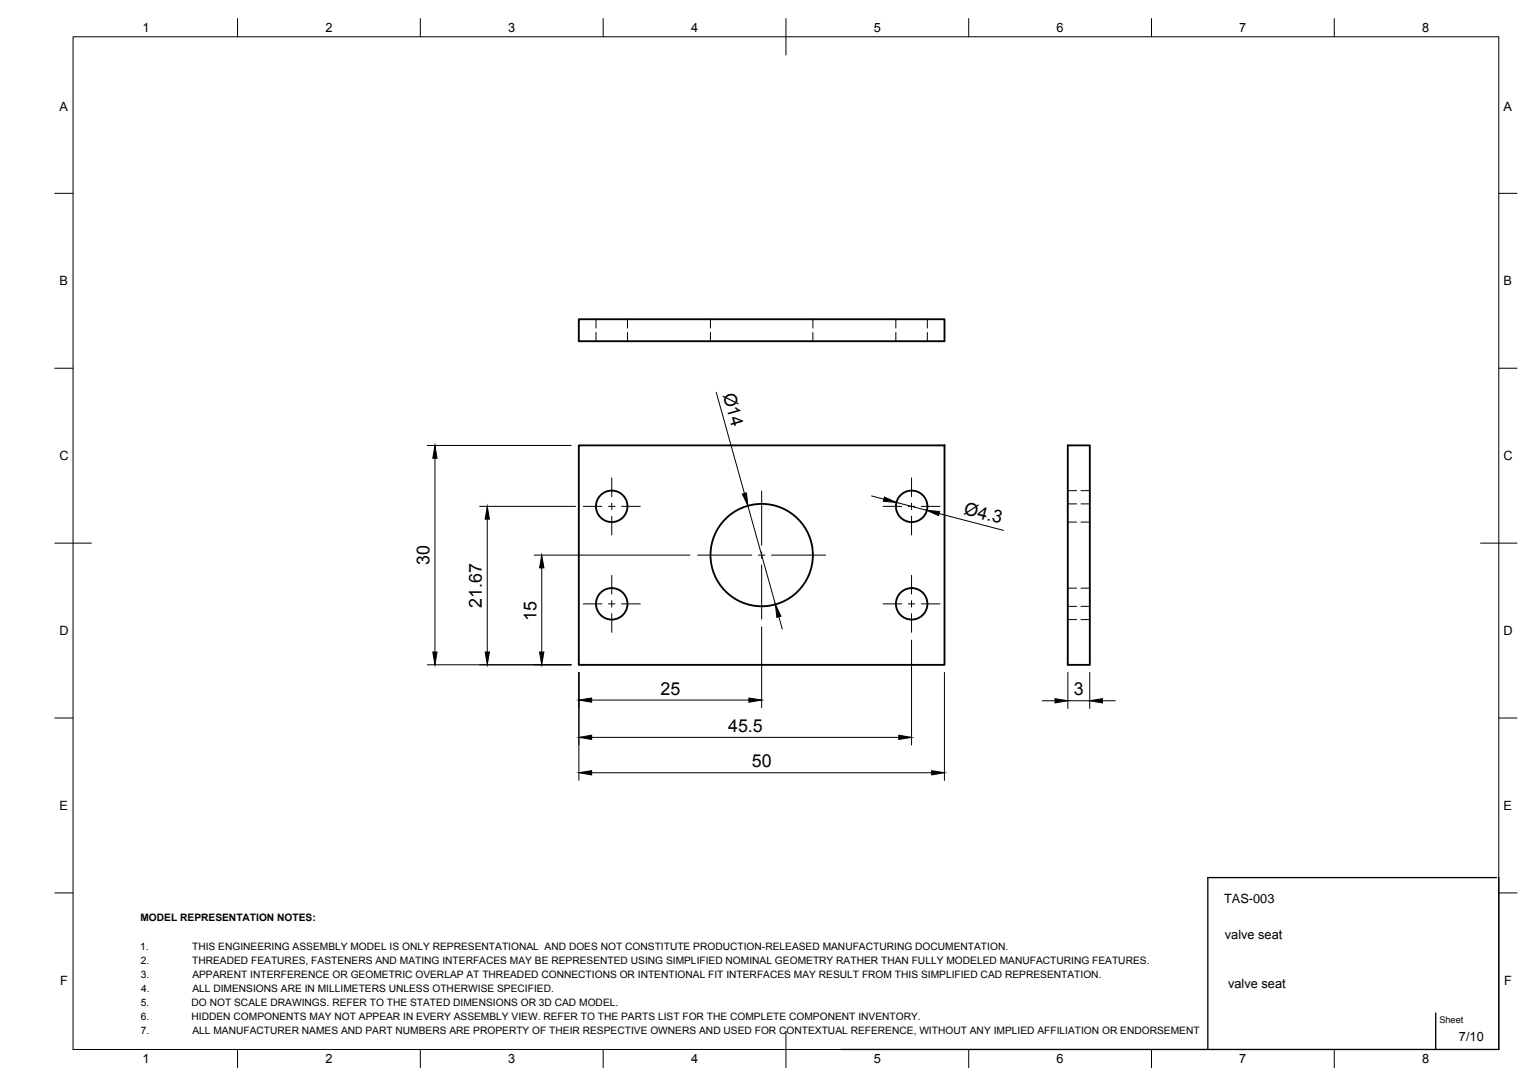
ISO-10303-21;
HEADER;
/* Generated by software containing ST-Developer
 * from STEP Tools, Inc. (www.steptools.com) 
 */

FILE_DESCRIPTION(
/* description */ ('STEP AP214'),
/* implementation_level */ '2;1');

FILE_NAME(
/* name */ 'valve seat.step',
/* time_stamp */ '2026-11-04T19:43:37-08:00',
/* author */ (''),
/* organization */ (''),
/* preprocessor_version */ 'ST-DEVELOPER v20.2',
/* originating_system */ 'Autodesk Translation Framework v15.17.0.0',
/* authorisation */ '');

FILE_SCHEMA (('AUTOMOTIVE_DESIGN { 1 0 10303 214 3 1 1 }'));
ENDSEC;

DATA;
#10=MECHANICAL_DESIGN_GEOMETRIC_PRESENTATION_REPRESENTATION('',(#119),#7627);
#101=SHAPE_REPRESENTATION_RELATIONSHIP('SRR','None',#7669,#110);
#110=ADVANCED_BREP_SHAPE_REPRESENTATION('',(#140),#7622);
#119=STYLED_ITEM('',(#7720),#140);
#140=MANIFOLD_SOLID_BREP('Body1',#2417);
#168=FACE_BOUND('',#518,.T.);
#169=FACE_BOUND('',#519,.T.);
#170=FACE_BOUND('',#520,.T.);
#171=FACE_BOUND('',#521,.T.);
#172=FACE_BOUND('',#522,.T.);
#173=FACE_BOUND('',#524,.T.);
#174=FACE_BOUND('',#525,.T.);
#175=FACE_BOUND('',#526,.T.);
#176=FACE_BOUND('',#527,.T.);
#177=FACE_BOUND('',#528,.T.);
#211=PLANE('',#2624);
#212=PLANE('',#2625);
#213=PLANE('',#2626);
#214=PLANE('',#2627);
#215=PLANE('',#2628);
#216=PLANE('',#2629);
#268=CYLINDRICAL_SURFACE('',#2609,2.15);
#269=CYLINDRICAL_SURFACE('',#2612,2.15);
#270=CYLINDRICAL_SURFACE('',#2615,2.15);
#271=CYLINDRICAL_SURFACE('',#2618,2.15);
#272=CYLINDRICAL_SURFACE('',#2621,7.);
#347=FACE_OUTER_BOUND('',#512,.T.);
#348=FACE_OUTER_BOUND('',#513,.T.);
#349=FACE_OUTER_BOUND('',#514,.T.);
#350=FACE_OUTER_BOUND('',#515,.T.);
#351=FACE_OUTER_BOUND('',#516,.T.);
#352=FACE_OUTER_BOUND('',#517,.T.);
#353=FACE_OUTER_BOUND('',#523,.T.);
#354=FACE_OUTER_BOUND('',#529,.T.);
#355=FACE_OUTER_BOUND('',#530,.T.);
#356=FACE_OUTER_BOUND('',#531,.T.);
#357=FACE_OUTER_BOUND('',#532,.T.);
#512=EDGE_LOOP('',(#1765,#1766,#1767,#1768));
#513=EDGE_LOOP('',(#1769,#1770,#1771,#1772));
#514=EDGE_LOOP('',(#1773,#1774,#1775,#1776));
#515=EDGE_LOOP('',(#1777,#1778,#1779,#1780));
#516=EDGE_LOOP('',(#1781,#1782,#1783,#1784));
#517=EDGE_LOOP('',(#1785,#1786,#1787,#1788));
#518=EDGE_LOOP('',(#1789));
#519=EDGE_LOOP('',(#1790));
#520=EDGE_LOOP('',(#1791));
#521=EDGE_LOOP('',(#1792));
#522=EDGE_LOOP('',(#1793));
#523=EDGE_LOOP('',(#1794,#1795,#1796,#1797));
#524=EDGE_LOOP('',(#1798));
#525=EDGE_LOOP('',(#1799));
#526=EDGE_LOOP('',(#1800));
#527=EDGE_LOOP('',(#1801));
#528=EDGE_LOOP('',(#1802));
#529=EDGE_LOOP('',(#1803,#1804,#1805,#1806));
#530=EDGE_LOOP('',(#1807,#1808,#1809,#1810));
#531=EDGE_LOOP('',(#1811,#1812,#1813,#1814));
#532=EDGE_LOOP('',(#1815,#1816,#1817,#1818));
#679=CIRCLE('',#2610,2.15);
#680=CIRCLE('',#2611,2.15);
#681=CIRCLE('',#2613,2.15);
#682=CIRCLE('',#2614,2.15);
#683=CIRCLE('',#2616,2.15);
#684=CIRCLE('',#2617,2.15);
#685=CIRCLE('',#2619,2.15);
#686=CIRCLE('',#2620,2.15);
#687=CIRCLE('',#2622,7.);
#688=CIRCLE('',#2623,7.);
#839=LINE('',#7093,#995);
#840=LINE('',#7099,#996);
#841=LINE('',#7105,#997);
#842=LINE('',#7111,#998);
#843=LINE('',#7117,#999);
#844=LINE('',#7122,#1000);
#845=LINE('',#7124,#1001);
#846=LINE('',#7126,#1002);
#847=LINE('',#7127,#1003);
#848=LINE('',#7131,#1004);
#849=LINE('',#7133,#1005);
#850=LINE('',#7135,#1006);
#851=LINE('',#7136,#1007);
#852=LINE('',#7138,#1008);
#853=LINE('',#7139,#1009);
#854=LINE('',#7141,#1010);
#855=LINE('',#7143,#1011);
#995=VECTOR('',#3054,2.15);
#996=VECTOR('',#3061,2.15);
#997=VECTOR('',#3068,2.15);
#998=VECTOR('',#3075,2.15);
#999=VECTOR('',#3082,7.);
#1000=VECTOR('',#3087,1000.);
#1001=VECTOR('',#3088,1000.);
#1002=VECTOR('',#3089,1000.);
#1003=VECTOR('',#3090,1000.);
#1004=VECTOR('',#3093,1000.);
#1005=VECTOR('',#3094,1000.);
#1006=VECTOR('',#3095,1000.);
#1007=VECTOR('',#3096,1000.);
#1008=VECTOR('',#3099,1000.);
#1009=VECTOR('',#3100,1000.);
#1010=VECTOR('',#3103,1000.);
#1011=VECTOR('',#3106,1000.);
#1163=VERTEX_POINT('',#7090);
#1164=VERTEX_POINT('',#7092);
#1165=VERTEX_POINT('',#7096);
#1166=VERTEX_POINT('',#7098);
#1167=VERTEX_POINT('',#7102);
#1168=VERTEX_POINT('',#7104);
#1169=VERTEX_POINT('',#7108);
#1170=VERTEX_POINT('',#7110);
#1171=VERTEX_POINT('',#7114);
#1172=VERTEX_POINT('',#7116);
#1173=VERTEX_POINT('',#7120);
#1174=VERTEX_POINT('',#7121);
#1175=VERTEX_POINT('',#7123);
#1176=VERTEX_POINT('',#7125);
#1177=VERTEX_POINT('',#7129);
#1178=VERTEX_POINT('',#7130);
#1179=VERTEX_POINT('',#7132);
#1180=VERTEX_POINT('',#7134);
#1377=EDGE_CURVE('',#1163,#1163,#679,.T.);
#1378=EDGE_CURVE('',#1163,#1164,#839,.T.);
#1379=EDGE_CURVE('',#1164,#1164,#680,.T.);
#1380=EDGE_CURVE('',#1165,#1165,#681,.T.);
#1381=EDGE_CURVE('',#1165,#1166,#840,.T.);
#1382=EDGE_CURVE('',#1166,#1166,#682,.T.);
#1383=EDGE_CURVE('',#1167,#1167,#683,.T.);
#1384=EDGE_CURVE('',#1167,#1168,#841,.T.);
#1385=EDGE_CURVE('',#1168,#1168,#684,.T.);
#1386=EDGE_CURVE('',#1169,#1169,#685,.T.);
#1387=EDGE_CURVE('',#1169,#1170,#842,.T.);
#1388=EDGE_CURVE('',#1170,#1170,#686,.T.);
#1389=EDGE_CURVE('',#1171,#1171,#687,.T.);
#1390=EDGE_CURVE('',#1171,#1172,#843,.T.);
#1391=EDGE_CURVE('',#1172,#1172,#688,.T.);
#1392=EDGE_CURVE('',#1173,#1174,#844,.T.);
#1393=EDGE_CURVE('',#1175,#1173,#845,.T.);
#1394=EDGE_CURVE('',#1176,#1175,#846,.T.);
#1395=EDGE_CURVE('',#1174,#1176,#847,.T.);
#1396=EDGE_CURVE('',#1177,#1178,#848,.T.);
#1397=EDGE_CURVE('',#1178,#1179,#849,.T.);
#1398=EDGE_CURVE('',#1179,#1180,#850,.T.);
#1399=EDGE_CURVE('',#1180,#1177,#851,.T.);
#1400=EDGE_CURVE('',#1178,#1174,#852,.T.);
#1401=EDGE_CURVE('',#1177,#1173,#853,.T.);
#1402=EDGE_CURVE('',#1179,#1176,#854,.T.);
#1403=EDGE_CURVE('',#1180,#1175,#855,.T.);
#1765=ORIENTED_EDGE('',*,*,#1377,.F.);
#1766=ORIENTED_EDGE('',*,*,#1378,.T.);
#1767=ORIENTED_EDGE('',*,*,#1379,.F.);
#1768=ORIENTED_EDGE('',*,*,#1378,.F.);
#1769=ORIENTED_EDGE('',*,*,#1380,.F.);
#1770=ORIENTED_EDGE('',*,*,#1381,.T.);
#1771=ORIENTED_EDGE('',*,*,#1382,.F.);
#1772=ORIENTED_EDGE('',*,*,#1381,.F.);
#1773=ORIENTED_EDGE('',*,*,#1383,.F.);
#1774=ORIENTED_EDGE('',*,*,#1384,.T.);
#1775=ORIENTED_EDGE('',*,*,#1385,.F.);
#1776=ORIENTED_EDGE('',*,*,#1384,.F.);
#1777=ORIENTED_EDGE('',*,*,#1386,.F.);
#1778=ORIENTED_EDGE('',*,*,#1387,.T.);
#1779=ORIENTED_EDGE('',*,*,#1388,.F.);
#1780=ORIENTED_EDGE('',*,*,#1387,.F.);
#1781=ORIENTED_EDGE('',*,*,#1389,.T.);
#1782=ORIENTED_EDGE('',*,*,#1390,.T.);
#1783=ORIENTED_EDGE('',*,*,#1391,.F.);
#1784=ORIENTED_EDGE('',*,*,#1390,.F.);
#1785=ORIENTED_EDGE('',*,*,#1392,.F.);
#1786=ORIENTED_EDGE('',*,*,#1393,.F.);
#1787=ORIENTED_EDGE('',*,*,#1394,.F.);
#1788=ORIENTED_EDGE('',*,*,#1395,.F.);
#1789=ORIENTED_EDGE('',*,*,#1386,.T.);
#1790=ORIENTED_EDGE('',*,*,#1383,.T.);
#1791=ORIENTED_EDGE('',*,*,#1377,.T.);
#1792=ORIENTED_EDGE('',*,*,#1380,.T.);
#1793=ORIENTED_EDGE('',*,*,#1391,.T.);
#1794=ORIENTED_EDGE('',*,*,#1396,.T.);
#1795=ORIENTED_EDGE('',*,*,#1397,.T.);
#1796=ORIENTED_EDGE('',*,*,#1398,.T.);
#1797=ORIENTED_EDGE('',*,*,#1399,.T.);
#1798=ORIENTED_EDGE('',*,*,#1389,.F.);
#1799=ORIENTED_EDGE('',*,*,#1379,.T.);
#1800=ORIENTED_EDGE('',*,*,#1382,.T.);
#1801=ORIENTED_EDGE('',*,*,#1385,.T.);
#1802=ORIENTED_EDGE('',*,*,#1388,.T.);
#1803=ORIENTED_EDGE('',*,*,#1392,.T.);
#1804=ORIENTED_EDGE('',*,*,#1400,.F.);
#1805=ORIENTED_EDGE('',*,*,#1396,.F.);
#1806=ORIENTED_EDGE('',*,*,#1401,.T.);
#1807=ORIENTED_EDGE('',*,*,#1395,.T.);
#1808=ORIENTED_EDGE('',*,*,#1402,.F.);
#1809=ORIENTED_EDGE('',*,*,#1397,.F.);
#1810=ORIENTED_EDGE('',*,*,#1400,.T.);
#1811=ORIENTED_EDGE('',*,*,#1394,.T.);
#1812=ORIENTED_EDGE('',*,*,#1403,.F.);
#1813=ORIENTED_EDGE('',*,*,#1398,.F.);
#1814=ORIENTED_EDGE('',*,*,#1402,.T.);
#1815=ORIENTED_EDGE('',*,*,#1393,.T.);
#1816=ORIENTED_EDGE('',*,*,#1401,.F.);
#1817=ORIENTED_EDGE('',*,*,#1399,.F.);
#1818=ORIENTED_EDGE('',*,*,#1403,.T.);
#2298=ADVANCED_FACE('',(#347),#268,.F.);
#2299=ADVANCED_FACE('',(#348),#269,.F.);
#2300=ADVANCED_FACE('',(#349),#270,.F.);
#2301=ADVANCED_FACE('',(#350),#271,.F.);
#2302=ADVANCED_FACE('',(#351),#272,.F.);
#2303=ADVANCED_FACE('',(#352,#168,#169,#170,#171,#172),#211,.T.);
#2304=ADVANCED_FACE('',(#353,#173,#174,#175,#176,#177),#212,.F.);
#2305=ADVANCED_FACE('',(#354),#213,.F.);
#2306=ADVANCED_FACE('',(#355),#214,.F.);
#2307=ADVANCED_FACE('',(#356),#215,.F.);
#2308=ADVANCED_FACE('',(#357),#216,.F.);
#2417=CLOSED_SHELL('',(#2298,#2299,#2300,#2301,#2302,#2303,#2304,#2305,
#2306,#2307,#2308));
#2608=AXIS2_PLACEMENT_3D('',#7088,#3048,#3049);
#2609=AXIS2_PLACEMENT_3D('',#7089,#3050,#3051);
#2610=AXIS2_PLACEMENT_3D('',#7091,#3052,#3053);
#2611=AXIS2_PLACEMENT_3D('',#7094,#3055,#3056);
#2612=AXIS2_PLACEMENT_3D('',#7095,#3057,#3058);
#2613=AXIS2_PLACEMENT_3D('',#7097,#3059,#3060);
#2614=AXIS2_PLACEMENT_3D('',#7100,#3062,#3063);
#2615=AXIS2_PLACEMENT_3D('',#7101,#3064,#3065);
#2616=AXIS2_PLACEMENT_3D('',#7103,#3066,#3067);
#2617=AXIS2_PLACEMENT_3D('',#7106,#3069,#3070);
#2618=AXIS2_PLACEMENT_3D('',#7107,#3071,#3072);
#2619=AXIS2_PLACEMENT_3D('',#7109,#3073,#3074);
#2620=AXIS2_PLACEMENT_3D('',#7112,#3076,#3077);
#2621=AXIS2_PLACEMENT_3D('',#7113,#3078,#3079);
#2622=AXIS2_PLACEMENT_3D('',#7115,#3080,#3081);
#2623=AXIS2_PLACEMENT_3D('',#7118,#3083,#3084);
#2624=AXIS2_PLACEMENT_3D('',#7119,#3085,#3086);
#2625=AXIS2_PLACEMENT_3D('',#7128,#3091,#3092);
#2626=AXIS2_PLACEMENT_3D('',#7137,#3097,#3098);
#2627=AXIS2_PLACEMENT_3D('',#7140,#3101,#3102);
#2628=AXIS2_PLACEMENT_3D('',#7142,#3104,#3105);
#2629=AXIS2_PLACEMENT_3D('',#7144,#3107,#3108);
#3048=DIRECTION('axis',(0.,0.,1.));
#3049=DIRECTION('refdir',(1.,0.,0.));
#3050=DIRECTION('center_axis',(0.,1.,0.));
#3051=DIRECTION('ref_axis',(0.,0.,1.));
#3052=DIRECTION('center_axis',(0.,1.,0.));
#3053=DIRECTION('ref_axis',(0.,0.,1.));
#3054=DIRECTION('',(0.,1.,0.));
#3055=DIRECTION('center_axis',(0.,-1.,0.));
#3056=DIRECTION('ref_axis',(0.,0.,-1.));
#3057=DIRECTION('center_axis',(0.,1.,0.));
#3058=DIRECTION('ref_axis',(0.,0.,1.));
#3059=DIRECTION('center_axis',(0.,1.,0.));
#3060=DIRECTION('ref_axis',(0.,0.,1.));
#3061=DIRECTION('',(0.,1.,0.));
#3062=DIRECTION('center_axis',(0.,-1.,0.));
#3063=DIRECTION('ref_axis',(0.,0.,-1.));
#3064=DIRECTION('center_axis',(0.,1.,0.));
#3065=DIRECTION('ref_axis',(0.,0.,1.));
#3066=DIRECTION('center_axis',(0.,1.,0.));
#3067=DIRECTION('ref_axis',(0.,0.,1.));
#3068=DIRECTION('',(0.,1.,0.));
#3069=DIRECTION('center_axis',(0.,-1.,0.));
#3070=DIRECTION('ref_axis',(0.,0.,-1.));
#3071=DIRECTION('center_axis',(0.,1.,0.));
#3072=DIRECTION('ref_axis',(0.,0.,1.));
#3073=DIRECTION('center_axis',(0.,1.,0.));
#3074=DIRECTION('ref_axis',(0.,0.,1.));
#3075=DIRECTION('',(0.,1.,0.));
#3076=DIRECTION('center_axis',(0.,-1.,0.));
#3077=DIRECTION('ref_axis',(0.,0.,-1.));
#3078=DIRECTION('center_axis',(0.,-1.,0.));
#3079=DIRECTION('ref_axis',(0.,0.,-1.));
#3080=DIRECTION('center_axis',(0.,1.,0.));
#3081=DIRECTION('ref_axis',(0.,0.,1.));
#3082=DIRECTION('',(0.,-1.,0.));
#3083=DIRECTION('center_axis',(0.,1.,0.));
#3084=DIRECTION('ref_axis',(0.,0.,1.));
#3085=DIRECTION('center_axis',(0.,-1.,0.));
#3086=DIRECTION('ref_axis',(0.,0.,-1.));
#3087=DIRECTION('',(0.,0.,-1.));
#3088=DIRECTION('',(1.,0.,0.));
#3089=DIRECTION('',(0.,0.,1.));
#3090=DIRECTION('',(-1.,0.,0.));
#3091=DIRECTION('center_axis',(0.,-1.,0.));
#3092=DIRECTION('ref_axis',(0.,0.,-1.));
#3093=DIRECTION('',(0.,0.,-1.));
#3094=DIRECTION('',(-1.,0.,0.));
#3095=DIRECTION('',(0.,0.,1.));
#3096=DIRECTION('',(1.,0.,0.));
#3097=DIRECTION('center_axis',(-1.,0.,0.));
#3098=DIRECTION('ref_axis',(0.,0.,1.));
#3099=DIRECTION('',(0.,-1.,0.));
#3100=DIRECTION('',(0.,-1.,0.));
#3101=DIRECTION('center_axis',(0.,0.,1.));
#3102=DIRECTION('ref_axis',(1.,0.,0.));
#3103=DIRECTION('',(0.,-1.,0.));
#3104=DIRECTION('center_axis',(1.,0.,0.));
#3105=DIRECTION('ref_axis',(0.,0.,-1.));
#3106=DIRECTION('',(0.,-1.,0.));
#3107=DIRECTION('center_axis',(0.,0.,-1.));
#3108=DIRECTION('ref_axis',(-1.,0.,0.));
#7088=CARTESIAN_POINT('',(0.,0.,0.));
#7089=CARTESIAN_POINT('Origin',(-6.66666666666667,15.,20.5));
#7090=CARTESIAN_POINT('',(-6.66666666666667,10.,18.35));
#7091=CARTESIAN_POINT('Origin',(-6.66666666666667,10.,20.5));
#7092=CARTESIAN_POINT('',(-6.66666666666667,13.,18.35));
#7093=CARTESIAN_POINT('',(-6.66666666666667,15.,18.35));
#7094=CARTESIAN_POINT('Origin',(-6.66666666666667,13.,20.5));
#7095=CARTESIAN_POINT('Origin',(6.66666666666666,15.,20.5));
#7096=CARTESIAN_POINT('',(6.66666666666666,10.,18.35));
#7097=CARTESIAN_POINT('Origin',(6.66666666666666,10.,20.5));
#7098=CARTESIAN_POINT('',(6.66666666666666,13.,18.35));
#7099=CARTESIAN_POINT('',(6.66666666666666,15.,18.35));
#7100=CARTESIAN_POINT('Origin',(6.66666666666666,13.,20.5));
#7101=CARTESIAN_POINT('Origin',(6.66666666666666,15.,-20.5));
#7102=CARTESIAN_POINT('',(6.66666666666666,10.,-22.65));
#7103=CARTESIAN_POINT('Origin',(6.66666666666666,10.,-20.5));
#7104=CARTESIAN_POINT('',(6.66666666666666,13.,-22.65));
#7105=CARTESIAN_POINT('',(6.66666666666666,15.,-22.65));
#7106=CARTESIAN_POINT('Origin',(6.66666666666666,13.,-20.5));
#7107=CARTESIAN_POINT('Origin',(-6.66666666666667,15.,-20.5));
#7108=CARTESIAN_POINT('',(-6.66666666666667,10.,-22.65));
#7109=CARTESIAN_POINT('Origin',(-6.66666666666667,10.,-20.5));
#7110=CARTESIAN_POINT('',(-6.66666666666667,13.,-22.65));
#7111=CARTESIAN_POINT('',(-6.66666666666667,15.,-22.65));
#7112=CARTESIAN_POINT('Origin',(-6.66666666666667,13.,-20.5));
#7113=CARTESIAN_POINT('Origin',(8.67361737988404E-15,13.,3.46944695195361E-15));
#7114=CARTESIAN_POINT('',(7.81636462048089E-15,13.,7.));
#7115=CARTESIAN_POINT('Origin',(8.67361737988404E-15,13.,3.46944695195361E-15));
#7116=CARTESIAN_POINT('',(7.81636462048089E-15,10.,7.));
#7117=CARTESIAN_POINT('',(7.81636462048089E-15,13.,7.));
#7118=CARTESIAN_POINT('Origin',(8.67361737988404E-15,10.,3.46944695195361E-15));
#7119=CARTESIAN_POINT('Origin',(0.,10.,0.));
#7120=CARTESIAN_POINT('',(15.,10.,25.));
#7121=CARTESIAN_POINT('',(15.,10.,-25.));
#7122=CARTESIAN_POINT('',(15.,10.,25.));
#7123=CARTESIAN_POINT('',(-15.,10.,25.));
#7124=CARTESIAN_POINT('',(-15.,10.,25.));
#7125=CARTESIAN_POINT('',(-15.,10.,-25.));
#7126=CARTESIAN_POINT('',(-15.,10.,25.));
#7127=CARTESIAN_POINT('',(-15.,10.,-25.));
#7128=CARTESIAN_POINT('Origin',(0.,13.,0.));
#7129=CARTESIAN_POINT('',(15.,13.,25.));
#7130=CARTESIAN_POINT('',(15.,13.,-25.));
#7131=CARTESIAN_POINT('',(15.,13.,25.));
#7132=CARTESIAN_POINT('',(-15.,13.,-25.));
#7133=CARTESIAN_POINT('',(-15.,13.,-25.));
#7134=CARTESIAN_POINT('',(-15.,13.,25.));
#7135=CARTESIAN_POINT('',(-15.,13.,25.));
#7136=CARTESIAN_POINT('',(-15.,13.,25.));
#7137=CARTESIAN_POINT('Origin',(15.,13.,25.));
#7138=CARTESIAN_POINT('',(15.,13.,-25.));
#7139=CARTESIAN_POINT('',(15.,13.,25.));
#7140=CARTESIAN_POINT('Origin',(-15.,13.,-25.));
#7141=CARTESIAN_POINT('',(-15.,13.,-25.));
#7142=CARTESIAN_POINT('Origin',(-15.,13.,25.));
#7143=CARTESIAN_POINT('',(-15.,13.,25.));
#7144=CARTESIAN_POINT('Origin',(-15.,13.,25.));
#7611=UNCERTAINTY_MEASURE_WITH_UNIT(LENGTH_MEASURE(0.01),#7628,
'DISTANCE_ACCURACY_VALUE',
'Maximum model space distance between geometric entities at asserted c
onnectivities');
#7616=UNCERTAINTY_MEASURE_WITH_UNIT(LENGTH_MEASURE(0.01),#7628,
'DISTANCE_ACCURACY_VALUE',
'Maximum model space distance between geometric entities at asserted c
onnectivities');
#7622=(
GEOMETRIC_REPRESENTATION_CONTEXT(3)
GLOBAL_UNCERTAINTY_ASSIGNED_CONTEXT((#7611))
GLOBAL_UNIT_ASSIGNED_CONTEXT((#7628,#7630,#7631))
REPRESENTATION_CONTEXT('','3D')
);
#7627=(
GEOMETRIC_REPRESENTATION_CONTEXT(3)
GLOBAL_UNCERTAINTY_ASSIGNED_CONTEXT((#7616))
GLOBAL_UNIT_ASSIGNED_CONTEXT((#7628,#7630,#7631))
REPRESENTATION_CONTEXT('','3D')
);
#7628=(
LENGTH_UNIT()
NAMED_UNIT(*)
SI_UNIT(.MILLI.,.METRE.)
);
#7630=(
NAMED_UNIT(*)
PLANE_ANGLE_UNIT()
SI_UNIT($,.RADIAN.)
);
#7631=(
NAMED_UNIT(*)
SI_UNIT($,.STERADIAN.)
SOLID_ANGLE_UNIT()
);
#7637=SHAPE_DEFINITION_REPRESENTATION(#7647,#7669);
#7647=PRODUCT_DEFINITION_SHAPE('',$,#7680);
#7669=SHAPE_REPRESENTATION('',(#2608),#7622);
#7674=PRODUCT_DEFINITION_CONTEXT('part definition',#7706,'design');
#7680=PRODUCT_DEFINITION('valve seat','valve seat',#7690,#7674);
#7690=PRODUCT_DEFINITION_FORMATION('',$,#7713);
#7706=APPLICATION_CONTEXT(
'Core Data for Automotive Mechanical Design Process');
#7707=PRODUCT_CONTEXT('part definition',#7706,'mechanical');
#7713=PRODUCT('valve seat','valve seat',$,(#7707));
#7720=PRESENTATION_STYLE_ASSIGNMENT((#7726));
#7726=SURFACE_STYLE_USAGE(.BOTH.,#7732);
#7732=SURFACE_SIDE_STYLE('',(#7738));
#7738=SURFACE_STYLE_FILL_AREA(#7744);
#7744=FILL_AREA_STYLE('Opaque(227,224,212)',(#7750));
#7750=FILL_AREA_STYLE_COLOUR('Opaque(227,224,212)',#7756);
#7756=COLOUR_RGB('Opaque(227,224,212)',0.890196078431372,0.87843137254902,
0.831372549019608);
ENDSEC;
END-ISO-10303-21;
